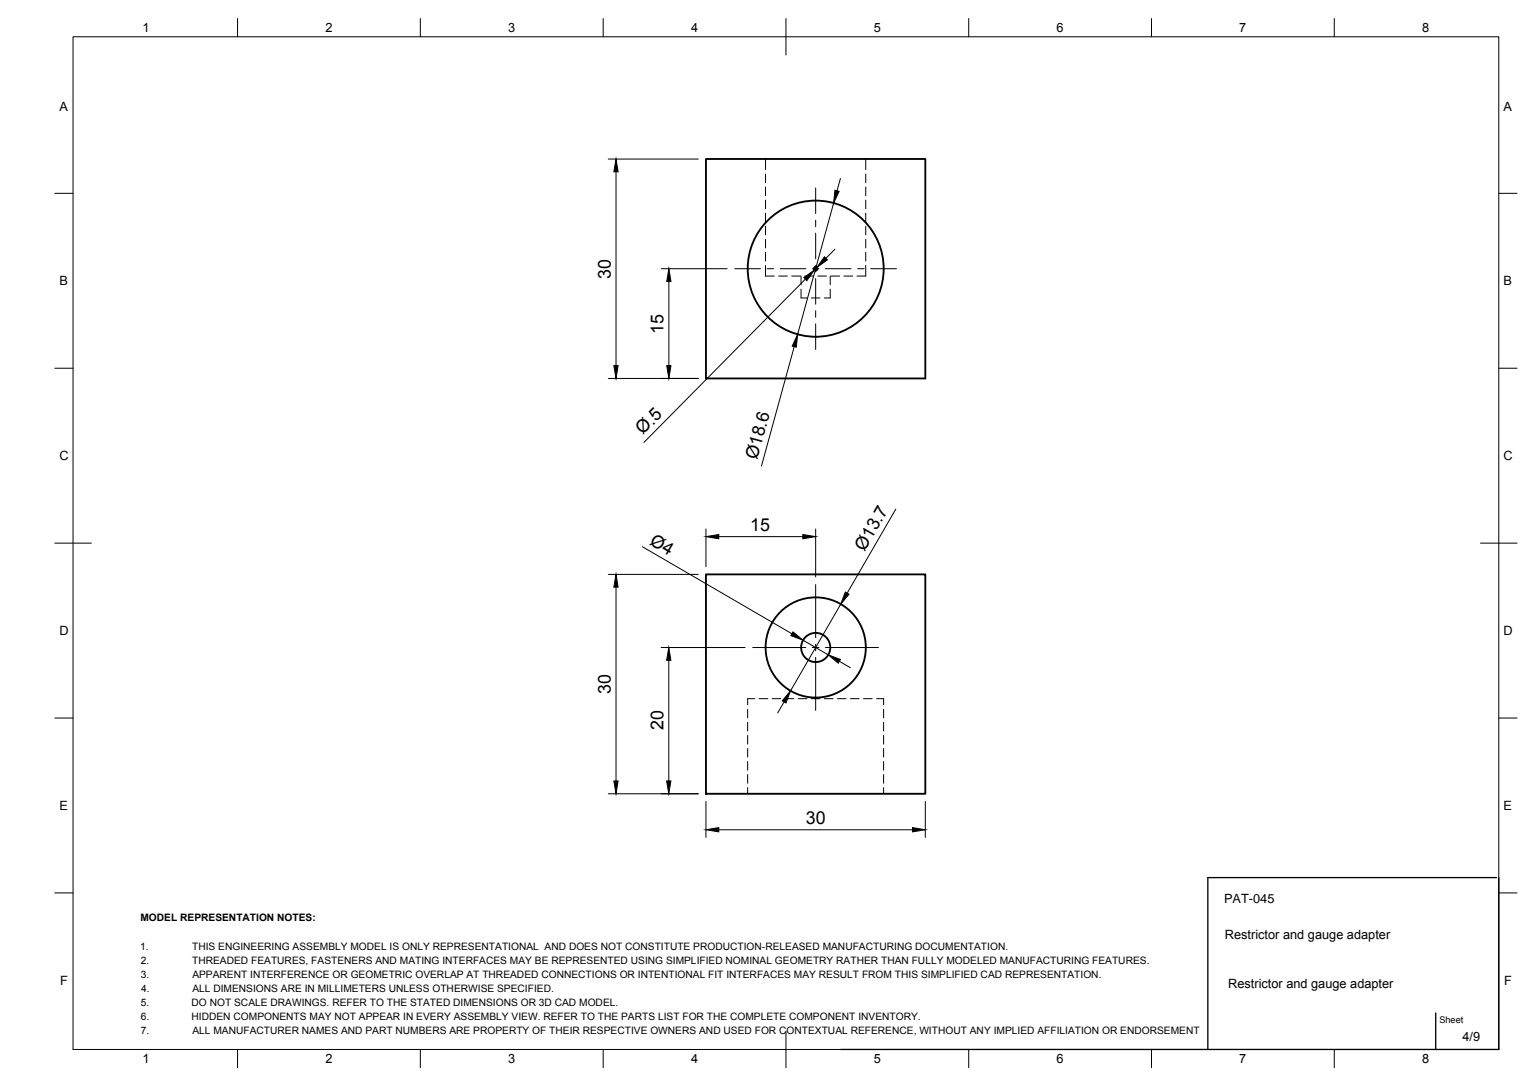
ISO-10303-21;
HEADER;
/* Generated by software containing ST-Developer
 * from STEP Tools, Inc. (www.steptools.com) 
 */

FILE_DESCRIPTION(
/* description */ ('Gauge isolation and snubber set'),
/* implementation_level */ '2;1');

FILE_NAME(
/* name */ 'Restrictor and gauge adapter.step',
/* time_stamp */ '2026-10-29T16:58:15-07:00',
/* author */ (''),
/* organization */ (''),
/* preprocessor_version */ 'ST-DEVELOPER v20.2',
/* originating_system */ 'Autodesk Translation Framework v15.17.0.0',
/* authorisation */ '');

FILE_SCHEMA (('AUTOMOTIVE_DESIGN { 1 0 10303 214 3 1 1 }'));
ENDSEC;

DATA;
#10=MECHANICAL_DESIGN_GEOMETRIC_PRESENTATION_REPRESENTATION('',(#93),#4043);
#77=SHAPE_REPRESENTATION_RELATIONSHIP('SRR','None',#4084,#85);
#85=ADVANCED_BREP_SHAPE_REPRESENTATION('',(#103),#4036);
#93=STYLED_ITEM('',(#4183),#103);
#103=MANIFOLD_SOLID_BREP('Body1',#2210);
#124=FACE_BOUND('',#415,.T.);
#125=FACE_BOUND('',#419,.T.);
#126=FACE_BOUND('',#423,.T.);
#127=FACE_BOUND('',#425,.T.);
#156=B_SPLINE_CURVE_WITH_KNOTS('',3,(#3445,#3446,#3447,#3448,#3449,#3450,
#3451,#3452,#3453,#3454),.UNSPECIFIED.,.F.,.F.,(4,2,2,2,4),(0.0753445150177796,
0.0847625796770749,0.0941806443363702,0.10359870843152,0.113016772526669),
 .UNSPECIFIED.);
#157=B_SPLINE_CURVE_WITH_KNOTS('',3,(#3456,#3457,#3458,#3459,#3460,#3461,
#3462,#3463,#3464,#3465),.UNSPECIFIED.,.F.,.F.,(4,2,2,2,4),(0.0376722575088898,
0.0470903216040394,0.056508385699189,0.0659264503584843,0.0753445150177796),
 .UNSPECIFIED.);
#158=B_SPLINE_CURVE_WITH_KNOTS('',3,(#3470,#3471,#3472,#3473,#3474,#3475,
#3476,#3477,#3478,#3479),.UNSPECIFIED.,.F.,.F.,(4,2,2,2,4),(0.,0.0094180646592953,
0.0188361293185906,0.0282541934137402,0.0376722575088898),.UNSPECIFIED.);
#159=B_SPLINE_CURVE_WITH_KNOTS('',3,(#3480,#3481,#3482,#3483,#3484,#3485,
#3486,#3487,#3488,#3489),.UNSPECIFIED.,.F.,.F.,(4,2,2,2,4),(0.113016772526669,
0.122434836621819,0.131852900716969,0.141270965376264,0.150689030035559),
 .UNSPECIFIED.);
#184=PLANE('',#2383);
#185=PLANE('',#2387);
#186=PLANE('',#2393);
#187=PLANE('',#2394);
#188=PLANE('',#2395);
#189=PLANE('',#2396);
#190=PLANE('',#2397);
#191=PLANE('',#2398);
#192=PLANE('',#2399);
#275=FACE_OUTER_BOUND('',#411,.T.);
#276=FACE_OUTER_BOUND('',#412,.T.);
#277=FACE_OUTER_BOUND('',#413,.T.);
#278=FACE_OUTER_BOUND('',#414,.T.);
#279=FACE_OUTER_BOUND('',#416,.T.);
#280=FACE_OUTER_BOUND('',#417,.T.);
#281=FACE_OUTER_BOUND('',#418,.T.);
#282=FACE_OUTER_BOUND('',#420,.T.);
#283=FACE_OUTER_BOUND('',#421,.T.);
#284=FACE_OUTER_BOUND('',#422,.T.);
#285=FACE_OUTER_BOUND('',#424,.T.);
#286=FACE_OUTER_BOUND('',#426,.T.);
#287=FACE_OUTER_BOUND('',#427,.T.);
#411=EDGE_LOOP('',(#1603,#1604,#1605,#1606));
#412=EDGE_LOOP('',(#1607));
#413=EDGE_LOOP('',(#1608,#1609,#1610,#1611,#1612,#1613,#1614,#1615,#1616,
#1617));
#414=EDGE_LOOP('',(#1618));
#415=EDGE_LOOP('',(#1619));
#416=EDGE_LOOP('',(#1620,#1621,#1622,#1623,#1624,#1625,#1626));
#417=EDGE_LOOP('',(#1627,#1628,#1629,#1630));
#418=EDGE_LOOP('',(#1631));
#419=EDGE_LOOP('',(#1632));
#420=EDGE_LOOP('',(#1633,#1634,#1635,#1636));
#421=EDGE_LOOP('',(#1637,#1638,#1639,#1640));
#422=EDGE_LOOP('',(#1641,#1642,#1643,#1644));
#423=EDGE_LOOP('',(#1645));
#424=EDGE_LOOP('',(#1646,#1647,#1648,#1649));
#425=EDGE_LOOP('',(#1650));
#426=EDGE_LOOP('',(#1651,#1652,#1653,#1654));
#427=EDGE_LOOP('',(#1655,#1656,#1657,#1658));
#564=CIRCLE('',#2381,0.199999999999999);
#565=CIRCLE('',#2382,0.199999999999999);
#566=CIRCLE('',#2385,0.685);
#567=CIRCLE('',#2386,0.685);
#568=CIRCLE('',#2389,0.0250000000000004);
#569=CIRCLE('',#2391,0.93);
#570=CIRCLE('',#2392,0.93);
#668=LINE('',#3436,#839);
#669=LINE('',#3443,#840);
#670=LINE('',#3467,#841);
#671=LINE('',#3494,#842);
#672=LINE('',#3499,#843);
#673=LINE('',#3505,#844);
#674=LINE('',#3507,#845);
#675=LINE('',#3509,#846);
#676=LINE('',#3510,#847);
#677=LINE('',#3513,#848);
#678=LINE('',#3515,#849);
#679=LINE('',#3516,#850);
#680=LINE('',#3519,#851);
#681=LINE('',#3521,#852);
#682=LINE('',#3522,#853);
#683=LINE('',#3524,#854);
#684=LINE('',#3525,#855);
#839=VECTOR('',#2741,0.199999999999999);
#840=VECTOR('',#2750,0.685);
#841=VECTOR('',#2751,0.685);
#842=VECTOR('',#2760,0.0250000000000004);
#843=VECTOR('',#2765,0.93);
#844=VECTOR('',#2772,1.);
#845=VECTOR('',#2773,1.);
#846=VECTOR('',#2774,1.);
#847=VECTOR('',#2775,1.);
#848=VECTOR('',#2778,1.);
#849=VECTOR('',#2779,1.);
#850=VECTOR('',#2780,1.);
#851=VECTOR('',#2783,1.);
#852=VECTOR('',#2784,1.);
#853=VECTOR('',#2785,1.);
#854=VECTOR('',#2788,1.);
#855=VECTOR('',#2789,1.);
#1023=VERTEX_POINT('',#3433);
#1024=VERTEX_POINT('',#3435);
#1025=VERTEX_POINT('',#3440);
#1026=VERTEX_POINT('',#3442);
#1027=VERTEX_POINT('',#3444);
#1028=VERTEX_POINT('',#3455);
#1029=VERTEX_POINT('',#3466);
#1030=VERTEX_POINT('',#3469);
#1031=VERTEX_POINT('',#3492);
#1032=VERTEX_POINT('',#3496);
#1033=VERTEX_POINT('',#3498);
#1034=VERTEX_POINT('',#3503);
#1035=VERTEX_POINT('',#3504);
#1036=VERTEX_POINT('',#3506);
#1037=VERTEX_POINT('',#3508);
#1038=VERTEX_POINT('',#3512);
#1039=VERTEX_POINT('',#3514);
#1040=VERTEX_POINT('',#3518);
#1041=VERTEX_POINT('',#3520);
#1240=EDGE_CURVE('',#1023,#1023,#564,.T.);
#1241=EDGE_CURVE('',#1023,#1024,#668,.T.);
#1242=EDGE_CURVE('',#1024,#1024,#565,.T.);
#1243=EDGE_CURVE('',#1025,#1025,#566,.T.);
#1244=EDGE_CURVE('',#1025,#1026,#669,.T.);
#1245=EDGE_CURVE('',#1027,#1026,#156,.T.);
#1246=EDGE_CURVE('',#1028,#1027,#157,.T.);
#1247=EDGE_CURVE('',#1028,#1029,#670,.T.);
#1248=EDGE_CURVE('',#1029,#1029,#567,.T.);
#1249=EDGE_CURVE('',#1030,#1028,#158,.T.);
#1250=EDGE_CURVE('',#1026,#1030,#159,.T.);
#1251=EDGE_CURVE('',#1031,#1031,#568,.T.);
#1252=EDGE_CURVE('',#1031,#1027,#671,.T.);
#1253=EDGE_CURVE('',#1032,#1032,#569,.T.);
#1254=EDGE_CURVE('',#1032,#1033,#672,.T.);
#1255=EDGE_CURVE('',#1033,#1033,#570,.T.);
#1256=EDGE_CURVE('',#1034,#1035,#673,.T.);
#1257=EDGE_CURVE('',#1035,#1036,#674,.T.);
#1258=EDGE_CURVE('',#1037,#1036,#675,.T.);
#1259=EDGE_CURVE('',#1034,#1037,#676,.T.);
#1260=EDGE_CURVE('',#1038,#1034,#677,.T.);
#1261=EDGE_CURVE('',#1039,#1037,#678,.T.);
#1262=EDGE_CURVE('',#1038,#1039,#679,.T.);
#1263=EDGE_CURVE('',#1040,#1038,#680,.T.);
#1264=EDGE_CURVE('',#1041,#1039,#681,.T.);
#1265=EDGE_CURVE('',#1040,#1041,#682,.T.);
#1266=EDGE_CURVE('',#1035,#1040,#683,.T.);
#1267=EDGE_CURVE('',#1036,#1041,#684,.T.);
#1603=ORIENTED_EDGE('',*,*,#1240,.F.);
#1604=ORIENTED_EDGE('',*,*,#1241,.T.);
#1605=ORIENTED_EDGE('',*,*,#1242,.T.);
#1606=ORIENTED_EDGE('',*,*,#1241,.F.);
#1607=ORIENTED_EDGE('',*,*,#1242,.F.);
#1608=ORIENTED_EDGE('',*,*,#1243,.F.);
#1609=ORIENTED_EDGE('',*,*,#1244,.T.);
#1610=ORIENTED_EDGE('',*,*,#1245,.F.);
#1611=ORIENTED_EDGE('',*,*,#1246,.F.);
#1612=ORIENTED_EDGE('',*,*,#1247,.T.);
#1613=ORIENTED_EDGE('',*,*,#1248,.T.);
#1614=ORIENTED_EDGE('',*,*,#1247,.F.);
#1615=ORIENTED_EDGE('',*,*,#1249,.F.);
#1616=ORIENTED_EDGE('',*,*,#1250,.F.);
#1617=ORIENTED_EDGE('',*,*,#1244,.F.);
#1618=ORIENTED_EDGE('',*,*,#1248,.F.);
#1619=ORIENTED_EDGE('',*,*,#1240,.T.);
#1620=ORIENTED_EDGE('',*,*,#1251,.F.);
#1621=ORIENTED_EDGE('',*,*,#1252,.T.);
#1622=ORIENTED_EDGE('',*,*,#1245,.T.);
#1623=ORIENTED_EDGE('',*,*,#1250,.T.);
#1624=ORIENTED_EDGE('',*,*,#1249,.T.);
#1625=ORIENTED_EDGE('',*,*,#1246,.T.);
#1626=ORIENTED_EDGE('',*,*,#1252,.F.);
#1627=ORIENTED_EDGE('',*,*,#1253,.F.);
#1628=ORIENTED_EDGE('',*,*,#1254,.T.);
#1629=ORIENTED_EDGE('',*,*,#1255,.T.);
#1630=ORIENTED_EDGE('',*,*,#1254,.F.);
#1631=ORIENTED_EDGE('',*,*,#1255,.F.);
#1632=ORIENTED_EDGE('',*,*,#1251,.T.);
#1633=ORIENTED_EDGE('',*,*,#1256,.T.);
#1634=ORIENTED_EDGE('',*,*,#1257,.T.);
#1635=ORIENTED_EDGE('',*,*,#1258,.F.);
#1636=ORIENTED_EDGE('',*,*,#1259,.F.);
#1637=ORIENTED_EDGE('',*,*,#1260,.T.);
#1638=ORIENTED_EDGE('',*,*,#1259,.T.);
#1639=ORIENTED_EDGE('',*,*,#1261,.F.);
#1640=ORIENTED_EDGE('',*,*,#1262,.F.);
#1641=ORIENTED_EDGE('',*,*,#1263,.T.);
#1642=ORIENTED_EDGE('',*,*,#1262,.T.);
#1643=ORIENTED_EDGE('',*,*,#1264,.F.);
#1644=ORIENTED_EDGE('',*,*,#1265,.F.);
#1645=ORIENTED_EDGE('',*,*,#1243,.T.);
#1646=ORIENTED_EDGE('',*,*,#1266,.T.);
#1647=ORIENTED_EDGE('',*,*,#1265,.T.);
#1648=ORIENTED_EDGE('',*,*,#1267,.F.);
#1649=ORIENTED_EDGE('',*,*,#1257,.F.);
#1650=ORIENTED_EDGE('',*,*,#1253,.T.);
#1651=ORIENTED_EDGE('',*,*,#1267,.T.);
#1652=ORIENTED_EDGE('',*,*,#1264,.T.);
#1653=ORIENTED_EDGE('',*,*,#1261,.T.);
#1654=ORIENTED_EDGE('',*,*,#1258,.T.);
#1655=ORIENTED_EDGE('',*,*,#1266,.F.);
#1656=ORIENTED_EDGE('',*,*,#1256,.F.);
#1657=ORIENTED_EDGE('',*,*,#1260,.F.);
#1658=ORIENTED_EDGE('',*,*,#1263,.F.);
#2059=CYLINDRICAL_SURFACE('',#2380,0.199999999999999);
#2060=CYLINDRICAL_SURFACE('',#2384,0.685);
#2061=CYLINDRICAL_SURFACE('',#2388,0.0250000000000004);
#2062=CYLINDRICAL_SURFACE('',#2390,0.93);
#2119=ADVANCED_FACE('',(#275),#2059,.F.);
#2120=ADVANCED_FACE('',(#276),#184,.F.);
#2121=ADVANCED_FACE('',(#277),#2060,.F.);
#2122=ADVANCED_FACE('',(#278,#124),#185,.F.);
#2123=ADVANCED_FACE('',(#279),#2061,.F.);
#2124=ADVANCED_FACE('',(#280),#2062,.F.);
#2125=ADVANCED_FACE('',(#281,#125),#186,.F.);
#2126=ADVANCED_FACE('',(#282),#187,.T.);
#2127=ADVANCED_FACE('',(#283),#188,.T.);
#2128=ADVANCED_FACE('',(#284,#126),#189,.T.);
#2129=ADVANCED_FACE('',(#285,#127),#190,.T.);
#2130=ADVANCED_FACE('',(#286),#191,.T.);
#2131=ADVANCED_FACE('',(#287),#192,.F.);
#2210=CLOSED_SHELL('',(#2119,#2120,#2121,#2122,#2123,#2124,#2125,#2126,
#2127,#2128,#2129,#2130,#2131));
#2379=AXIS2_PLACEMENT_3D('',#3431,#2735,#2736);
#2380=AXIS2_PLACEMENT_3D('',#3432,#2737,#2738);
#2381=AXIS2_PLACEMENT_3D('',#3434,#2739,#2740);
#2382=AXIS2_PLACEMENT_3D('',#3437,#2742,#2743);
#2383=AXIS2_PLACEMENT_3D('',#3438,#2744,#2745);
#2384=AXIS2_PLACEMENT_3D('',#3439,#2746,#2747);
#2385=AXIS2_PLACEMENT_3D('',#3441,#2748,#2749);
#2386=AXIS2_PLACEMENT_3D('',#3468,#2752,#2753);
#2387=AXIS2_PLACEMENT_3D('',#3490,#2754,#2755);
#2388=AXIS2_PLACEMENT_3D('',#3491,#2756,#2757);
#2389=AXIS2_PLACEMENT_3D('',#3493,#2758,#2759);
#2390=AXIS2_PLACEMENT_3D('',#3495,#2761,#2762);
#2391=AXIS2_PLACEMENT_3D('',#3497,#2763,#2764);
#2392=AXIS2_PLACEMENT_3D('',#3500,#2766,#2767);
#2393=AXIS2_PLACEMENT_3D('',#3501,#2768,#2769);
#2394=AXIS2_PLACEMENT_3D('',#3502,#2770,#2771);
#2395=AXIS2_PLACEMENT_3D('',#3511,#2776,#2777);
#2396=AXIS2_PLACEMENT_3D('',#3517,#2781,#2782);
#2397=AXIS2_PLACEMENT_3D('',#3523,#2786,#2787);
#2398=AXIS2_PLACEMENT_3D('',#3526,#2790,#2791);
#2399=AXIS2_PLACEMENT_3D('',#3527,#2792,#2793);
#2735=DIRECTION('axis',(0.,0.,1.));
#2736=DIRECTION('refdir',(1.,0.,0.));
#2737=DIRECTION('center_axis',(0.,1.,0.));
#2738=DIRECTION('ref_axis',(1.,0.,0.));
#2739=DIRECTION('center_axis',(0.,1.,0.));
#2740=DIRECTION('ref_axis',(1.,0.,0.));
#2741=DIRECTION('',(0.,1.,0.));
#2742=DIRECTION('center_axis',(0.,1.,0.));
#2743=DIRECTION('ref_axis',(1.,0.,0.));
#2744=DIRECTION('center_axis',(0.,1.,0.));
#2745=DIRECTION('ref_axis',(1.,0.,0.));
#2746=DIRECTION('center_axis',(0.,1.,0.));
#2747=DIRECTION('ref_axis',(1.,0.,0.));
#2748=DIRECTION('center_axis',(0.,1.,0.));
#2749=DIRECTION('ref_axis',(1.,0.,0.));
#2750=DIRECTION('',(0.,1.,0.));
#2751=DIRECTION('',(0.,1.,0.));
#2752=DIRECTION('center_axis',(0.,1.,0.));
#2753=DIRECTION('ref_axis',(1.,0.,0.));
#2754=DIRECTION('center_axis',(0.,1.,0.));
#2755=DIRECTION('ref_axis',(1.,0.,0.));
#2756=DIRECTION('center_axis',(1.,0.,0.));
#2757=DIRECTION('ref_axis',(0.,0.,-1.));
#2758=DIRECTION('center_axis',(1.,0.,0.));
#2759=DIRECTION('ref_axis',(0.,0.,-1.));
#2760=DIRECTION('',(1.,0.,0.));
#2761=DIRECTION('center_axis',(1.,0.,0.));
#2762=DIRECTION('ref_axis',(0.,0.,-1.));
#2763=DIRECTION('center_axis',(1.,0.,0.));
#2764=DIRECTION('ref_axis',(0.,0.,-1.));
#2765=DIRECTION('',(1.,0.,0.));
#2766=DIRECTION('center_axis',(1.,0.,0.));
#2767=DIRECTION('ref_axis',(0.,0.,-1.));
#2768=DIRECTION('center_axis',(1.,0.,0.));
#2769=DIRECTION('ref_axis',(0.,0.,-1.));
#2770=DIRECTION('center_axis',(0.,1.,0.));
#2771=DIRECTION('ref_axis',(-1.,0.,0.));
#2772=DIRECTION('',(-1.,0.,0.));
#2773=DIRECTION('',(0.,0.,1.));
#2774=DIRECTION('',(-1.,0.,0.));
#2775=DIRECTION('',(0.,0.,1.));
#2776=DIRECTION('center_axis',(1.,0.,0.));
#2777=DIRECTION('ref_axis',(0.,1.,0.));
#2778=DIRECTION('',(0.,1.,0.));
#2779=DIRECTION('',(0.,1.,0.));
#2780=DIRECTION('',(0.,0.,1.));
#2781=DIRECTION('center_axis',(0.,-1.,0.));
#2782=DIRECTION('ref_axis',(1.,0.,0.));
#2783=DIRECTION('',(1.,0.,0.));
#2784=DIRECTION('',(1.,0.,0.));
#2785=DIRECTION('',(0.,0.,1.));
#2786=DIRECTION('center_axis',(-1.,0.,0.));
#2787=DIRECTION('ref_axis',(0.,-1.,0.));
#2788=DIRECTION('',(0.,-1.,0.));
#2789=DIRECTION('',(0.,-1.,0.));
#2790=DIRECTION('center_axis',(0.,0.,1.));
#2791=DIRECTION('ref_axis',(1.,0.,0.));
#2792=DIRECTION('center_axis',(0.,0.,1.));
#2793=DIRECTION('ref_axis',(1.,0.,0.));
#3431=CARTESIAN_POINT('',(0.,0.,0.));
#3432=CARTESIAN_POINT('Origin',(8.,0.,8.5));
#3433=CARTESIAN_POINT('',(7.8,0.1,8.5));
#3434=CARTESIAN_POINT('Origin',(8.,0.1,8.5));
#3435=CARTESIAN_POINT('',(7.8,0.4,8.5));
#3436=CARTESIAN_POINT('',(7.8,0.,8.5));
#3437=CARTESIAN_POINT('Origin',(8.,0.4,8.5));
#3438=CARTESIAN_POINT('Origin',(8.,0.4,8.5));
#3439=CARTESIAN_POINT('Origin',(8.,-1.6,8.5));
#3440=CARTESIAN_POINT('',(7.315,-1.5,8.5));
#3441=CARTESIAN_POINT('Origin',(8.,-1.5,8.5));
#3442=CARTESIAN_POINT('',(7.315,-0.0250000000000004,8.5));
#3443=CARTESIAN_POINT('',(7.315,-1.6,8.5));
#3444=CARTESIAN_POINT('',(7.31545635639501,-3.06161699786843E-18,8.525));
#3445=CARTESIAN_POINT('Ctrl Pts',(7.31545635639501,6.50521303742584E-19,
8.525));
#3446=CARTESIAN_POINT('Ctrl Pts',(7.31545635639501,-0.00313935488643177,
8.525));
#3447=CARTESIAN_POINT('Ctrl Pts',(7.31543253912522,-0.00648777233356316,
8.5243725421486));
#3448=CARTESIAN_POINT('Ctrl Pts',(7.31534646113093,-0.0126471731738094,
8.521821113914));
#3449=CARTESIAN_POINT('Ctrl Pts',(7.31528543721954,-0.0154581801568198,
8.51989715890251));
#3450=CARTESIAN_POINT('Ctrl Pts',(7.31517084314585,-0.0198971587695597,
8.51545818028977));
#3451=CARTESIAN_POINT('Ctrl Pts',(7.31510983697032,-0.0218211138748799,
8.51264717324355));
#3452=CARTESIAN_POINT('Ctrl Pts',(7.31502379952475,-0.0243725422072981,
8.50648777221657));
#3453=CARTESIAN_POINT('Ctrl Pts',(7.315,-0.0250000000000004,8.50313935469838));
#3454=CARTESIAN_POINT('Ctrl Pts',(7.315,-0.0250000000000004,8.5));
#3455=CARTESIAN_POINT('',(7.315,0.0250000000000004,8.5));
#3456=CARTESIAN_POINT('Ctrl Pts',(7.315,0.0250000000000004,8.5));
#3457=CARTESIAN_POINT('Ctrl Pts',(7.315,0.0250000000000004,8.50313935469838));
#3458=CARTESIAN_POINT('Ctrl Pts',(7.31502379952475,0.0243725422072981,8.50648777221657));
#3459=CARTESIAN_POINT('Ctrl Pts',(7.31510983697032,0.0218211138748799,8.51264717324355));
#3460=CARTESIAN_POINT('Ctrl Pts',(7.31517084314585,0.0198971587695597,8.51545818028977));
#3461=CARTESIAN_POINT('Ctrl Pts',(7.31528543721954,0.0154581801568198,8.51989715890251));
#3462=CARTESIAN_POINT('Ctrl Pts',(7.31534646113093,0.0126471731738094,8.521821113914));
#3463=CARTESIAN_POINT('Ctrl Pts',(7.31543253912522,0.00648777233356315,
8.5243725421486));
#3464=CARTESIAN_POINT('Ctrl Pts',(7.31545635639501,0.00313935488643177,
8.525));
#3465=CARTESIAN_POINT('Ctrl Pts',(7.31545635639501,6.50521303491303E-19,
8.525));
#3466=CARTESIAN_POINT('',(7.315,0.1,8.5));
#3467=CARTESIAN_POINT('',(7.315,-1.6,8.5));
#3468=CARTESIAN_POINT('Origin',(8.,0.1,8.5));
#3469=CARTESIAN_POINT('',(7.31545635639501,0.,8.475));
#3470=CARTESIAN_POINT('Ctrl Pts',(7.31545635639501,0.,8.475));
#3471=CARTESIAN_POINT('Ctrl Pts',(7.31545635639501,0.00313935488643177,
8.475));
#3472=CARTESIAN_POINT('Ctrl Pts',(7.31543253912522,0.00648777233356316,
8.4756274578514));
#3473=CARTESIAN_POINT('Ctrl Pts',(7.31534646113093,0.0126471731738094,8.478178886086));
#3474=CARTESIAN_POINT('Ctrl Pts',(7.31528543721954,0.0154581801568198,8.48010284109749));
#3475=CARTESIAN_POINT('Ctrl Pts',(7.31517084314585,0.0198971587695597,8.48454181971023));
#3476=CARTESIAN_POINT('Ctrl Pts',(7.31510983697032,0.0218211138748799,8.48735282675645));
#3477=CARTESIAN_POINT('Ctrl Pts',(7.31502379952475,0.0243725422072981,8.49351222778343));
#3478=CARTESIAN_POINT('Ctrl Pts',(7.315,0.0250000000000004,8.49686064530162));
#3479=CARTESIAN_POINT('Ctrl Pts',(7.315,0.0250000000000004,8.5));
#3480=CARTESIAN_POINT('Ctrl Pts',(7.315,-0.0250000000000004,8.5));
#3481=CARTESIAN_POINT('Ctrl Pts',(7.315,-0.0250000000000004,8.49686064530162));
#3482=CARTESIAN_POINT('Ctrl Pts',(7.31502379952475,-0.0243725422072981,
8.49351222778343));
#3483=CARTESIAN_POINT('Ctrl Pts',(7.31510983697032,-0.0218211138748799,
8.48735282675645));
#3484=CARTESIAN_POINT('Ctrl Pts',(7.31517084314585,-0.0198971587695597,
8.48454181971023));
#3485=CARTESIAN_POINT('Ctrl Pts',(7.31528543721954,-0.0154581801568198,
8.48010284109749));
#3486=CARTESIAN_POINT('Ctrl Pts',(7.31534646113093,-0.012647173173808,8.478178886086));
#3487=CARTESIAN_POINT('Ctrl Pts',(7.31543253912522,-0.00648777233356145,
8.4756274578514));
#3488=CARTESIAN_POINT('Ctrl Pts',(7.31545635639501,-0.00313935488643176,
8.475));
#3489=CARTESIAN_POINT('Ctrl Pts',(7.31545635639501,0.,8.475));
#3490=CARTESIAN_POINT('Origin',(8.,0.1,8.5));
#3491=CARTESIAN_POINT('Origin',(7.2,0.,8.5));
#3492=CARTESIAN_POINT('',(7.3,-3.06161699786843E-18,8.525));
#3493=CARTESIAN_POINT('Origin',(7.3,0.,8.5));
#3494=CARTESIAN_POINT('',(7.2,-3.06161699786843E-18,8.525));
#3495=CARTESIAN_POINT('Origin',(5.9,0.,8.5));
#3496=CARTESIAN_POINT('',(6.,-1.13892152320704E-16,9.43));
#3497=CARTESIAN_POINT('Origin',(6.,0.,8.5));
#3498=CARTESIAN_POINT('',(7.3,-1.13892152320704E-16,9.43));
#3499=CARTESIAN_POINT('',(5.9,-1.13892152320704E-16,9.43));
#3500=CARTESIAN_POINT('Origin',(7.3,0.,8.5));
#3501=CARTESIAN_POINT('Origin',(7.3,0.,8.5));
#3502=CARTESIAN_POINT('Origin',(9.,1.5,7.));
#3503=CARTESIAN_POINT('',(9.,1.5,7.));
#3504=CARTESIAN_POINT('',(6.,1.5,7.));
#3505=CARTESIAN_POINT('',(9.,1.5,7.));
#3506=CARTESIAN_POINT('',(6.,1.5,10.));
#3507=CARTESIAN_POINT('',(6.,1.5,7.));
#3508=CARTESIAN_POINT('',(9.,1.5,10.));
#3509=CARTESIAN_POINT('',(9.,1.5,10.));
#3510=CARTESIAN_POINT('',(9.,1.5,7.));
#3511=CARTESIAN_POINT('Origin',(9.,-1.5,7.));
#3512=CARTESIAN_POINT('',(9.,-1.5,7.));
#3513=CARTESIAN_POINT('',(9.,-1.5,7.));
#3514=CARTESIAN_POINT('',(9.,-1.5,10.));
#3515=CARTESIAN_POINT('',(9.,-1.5,10.));
#3516=CARTESIAN_POINT('',(9.,-1.5,7.));
#3517=CARTESIAN_POINT('Origin',(6.,-1.5,7.));
#3518=CARTESIAN_POINT('',(6.,-1.5,7.));
#3519=CARTESIAN_POINT('',(6.,-1.5,7.));
#3520=CARTESIAN_POINT('',(6.,-1.5,10.));
#3521=CARTESIAN_POINT('',(6.,-1.5,10.));
#3522=CARTESIAN_POINT('',(6.,-1.5,7.));
#3523=CARTESIAN_POINT('Origin',(6.,1.5,7.));
#3524=CARTESIAN_POINT('',(6.,1.5,7.));
#3525=CARTESIAN_POINT('',(6.,1.5,10.));
#3526=CARTESIAN_POINT('Origin',(7.5,0.,10.));
#3527=CARTESIAN_POINT('Origin',(7.5,0.,7.));
#4025=UNCERTAINTY_MEASURE_WITH_UNIT(LENGTH_MEASURE(0.001),#4044,
'DISTANCE_ACCURACY_VALUE',
'Maximum model space distance between geometric entities at asserted c
onnectivities');
#4032=UNCERTAINTY_MEASURE_WITH_UNIT(LENGTH_MEASURE(0.001),#4044,
'DISTANCE_ACCURACY_VALUE',
'Maximum model space distance between geometric entities at asserted c
onnectivities');
#4036=(
GEOMETRIC_REPRESENTATION_CONTEXT(3)
GLOBAL_UNCERTAINTY_ASSIGNED_CONTEXT((#4025))
GLOBAL_UNIT_ASSIGNED_CONTEXT((#4044,#4046,#4047))
REPRESENTATION_CONTEXT('','3D')
);
#4043=(
GEOMETRIC_REPRESENTATION_CONTEXT(3)
GLOBAL_UNCERTAINTY_ASSIGNED_CONTEXT((#4032))
GLOBAL_UNIT_ASSIGNED_CONTEXT((#4044,#4046,#4047))
REPRESENTATION_CONTEXT('','3D')
);
#4044=(
LENGTH_UNIT()
NAMED_UNIT(*)
SI_UNIT(.CENTI.,.METRE.)
);
#4046=(
NAMED_UNIT(*)
PLANE_ANGLE_UNIT()
SI_UNIT($,.RADIAN.)
);
#4047=(
NAMED_UNIT(*)
SI_UNIT($,.STERADIAN.)
SOLID_ANGLE_UNIT()
);
#4051=SHAPE_DEFINITION_REPRESENTATION(#4061,#4084);
#4061=PRODUCT_DEFINITION_SHAPE('',$,#4095);
#4084=SHAPE_REPRESENTATION('',(#2379),#4036);
#4091=PRODUCT_DEFINITION_CONTEXT('part definition',#4123,'design');
#4095=PRODUCT_DEFINITION('Restrictor and gauge adapter',
'Restrictor and gauge adapter',#4105,#4091);
#4105=PRODUCT_DEFINITION_FORMATION('',$,#4128);
#4123=APPLICATION_CONTEXT(
'Core Data for Automotive Mechanical Design Process');
#4124=PRODUCT_CONTEXT('part definition',#4123,'mechanical');
#4128=PRODUCT('Restrictor and gauge adapter',
'Restrictor and gauge adapter','Restrictor and gauge adapter',(#4124));
#4177=COLOUR_RGB('Light Blue',0.38,0.62,0.78);
#4178=FILL_AREA_STYLE_COLOUR('',#4177);
#4179=FILL_AREA_STYLE('',(#4178));
#4180=SURFACE_STYLE_FILL_AREA(#4179);
#4181=SURFACE_SIDE_STYLE('',(#4180));
#4182=SURFACE_STYLE_USAGE(.BOTH.,#4181);
#4183=PRESENTATION_STYLE_ASSIGNMENT((#4182));
ENDSEC;
END-ISO-10303-21;
